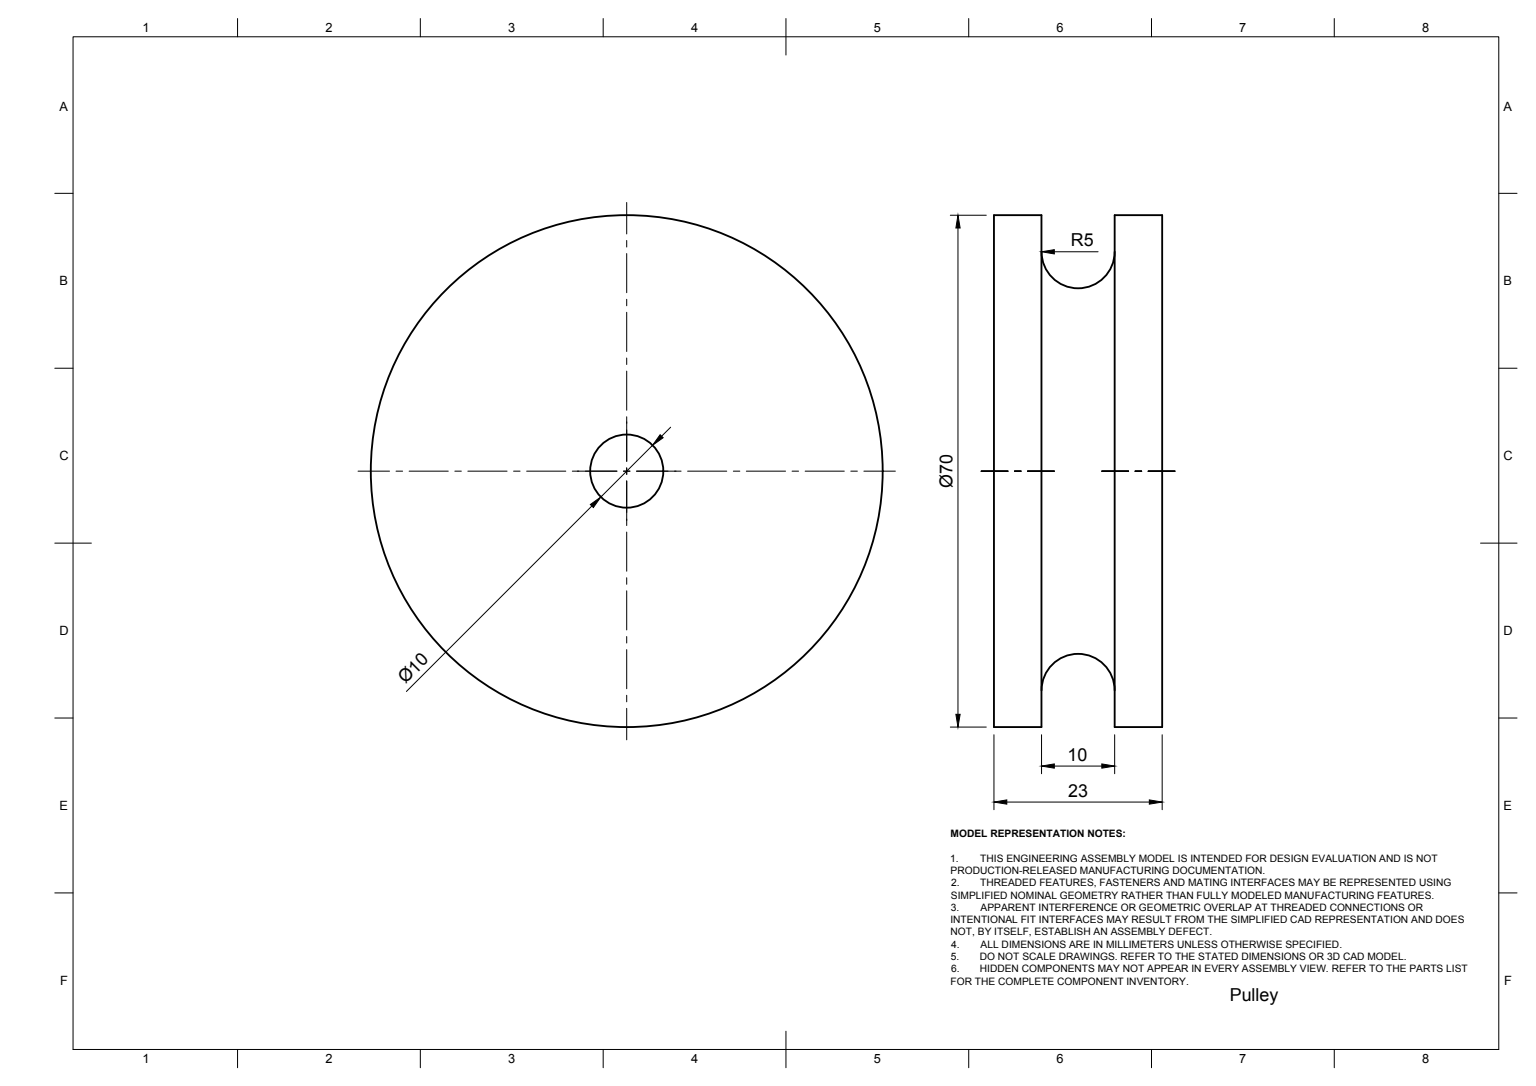
ISO-10303-21;
HEADER;
/* Generated by software containing ST-Developer
 * from STEP Tools, Inc. (www.steptools.com) 
 */

FILE_DESCRIPTION(
/* description */ (''),
/* implementation_level */ '2;1');

FILE_NAME(
/* name */ 'Pulley.step',
/* time_stamp */ '2026-10-07T11:02:43-07:00',
/* author */ (''),
/* organization */ (''),
/* preprocessor_version */ 'ST-DEVELOPER v20.2',
/* originating_system */ 'Autodesk Translation Framework v15.15.0.0',
/* authorisation */ '');

FILE_SCHEMA (('AUTOMOTIVE_DESIGN { 1 0 10303 214 3 1 1 }'));
ENDSEC;

DATA;
#10=MECHANICAL_DESIGN_GEOMETRIC_PRESENTATION_REPRESENTATION('',(#68),#5505);
#51=TOROIDAL_SURFACE('',#3505,30.,5.);
#54=SHAPE_REPRESENTATION_RELATIONSHIP('SRR','None',#5539,#61);
#61=ADVANCED_BREP_SHAPE_REPRESENTATION('',(#75),#5500);
#68=STYLED_ITEM('',(#5583),#75);
#75=MANIFOLD_SOLID_BREP('Body1',#3295);
#98=FACE_BOUND('',#504,.T.);
#99=FACE_BOUND('',#507,.T.);
#100=FACE_BOUND('',#510,.T.);
#101=FACE_BOUND('',#513,.T.);
#129=CYLINDRICAL_SURFACE('',#3496,5.);
#130=CYLINDRICAL_SURFACE('',#3501,35.);
#131=CYLINDRICAL_SURFACE('',#3510,35.);
#185=CIRCLE('',#3497,5.);
#186=CIRCLE('',#3498,5.);
#187=CIRCLE('',#3500,35.);
#188=CIRCLE('',#3502,35.);
#189=CIRCLE('',#3504,30.);
#190=CIRCLE('',#3506,5.);
#191=CIRCLE('',#3507,30.);
#192=CIRCLE('',#3509,35.);
#193=CIRCLE('',#3511,35.);
#318=FACE_OUTER_BOUND('',#502,.T.);
#319=FACE_OUTER_BOUND('',#503,.T.);
#320=FACE_OUTER_BOUND('',#505,.T.);
#321=FACE_OUTER_BOUND('',#506,.T.);
#322=FACE_OUTER_BOUND('',#508,.T.);
#323=FACE_OUTER_BOUND('',#509,.T.);
#324=FACE_OUTER_BOUND('',#511,.T.);
#325=FACE_OUTER_BOUND('',#512,.T.);
#502=EDGE_LOOP('',(#2576,#2577,#2578,#2579));
#503=EDGE_LOOP('',(#2580));
#504=EDGE_LOOP('',(#2581));
#505=EDGE_LOOP('',(#2582,#2583,#2584,#2585));
#506=EDGE_LOOP('',(#2586));
#507=EDGE_LOOP('',(#2587));
#508=EDGE_LOOP('',(#2588,#2589,#2590,#2591));
#509=EDGE_LOOP('',(#2592));
#510=EDGE_LOOP('',(#2593));
#511=EDGE_LOOP('',(#2594,#2595,#2596,#2597));
#512=EDGE_LOOP('',(#2598));
#513=EDGE_LOOP('',(#2599));
#809=LINE('',#5039,#1179);
#810=LINE('',#5046,#1180);
#811=LINE('',#5060,#1181);
#1179=VECTOR('',#4093,5.);
#1180=VECTOR('',#4102,35.);
#1181=VECTOR('',#4121,35.);
#1501=VERTEX_POINT('',#5036);
#1502=VERTEX_POINT('',#5038);
#1503=VERTEX_POINT('',#5042);
#1504=VERTEX_POINT('',#5045);
#1505=VERTEX_POINT('',#5049);
#1506=VERTEX_POINT('',#5052);
#1507=VERTEX_POINT('',#5056);
#1508=VERTEX_POINT('',#5059);
#1883=EDGE_CURVE('',#1501,#1501,#185,.T.);
#1884=EDGE_CURVE('',#1501,#1502,#809,.T.);
#1885=EDGE_CURVE('',#1502,#1502,#186,.T.);
#1886=EDGE_CURVE('',#1503,#1503,#187,.T.);
#1887=EDGE_CURVE('',#1503,#1504,#810,.T.);
#1888=EDGE_CURVE('',#1504,#1504,#188,.T.);
#1889=EDGE_CURVE('',#1505,#1505,#189,.T.);
#1890=EDGE_CURVE('',#1505,#1506,#190,.T.);
#1891=EDGE_CURVE('',#1506,#1506,#191,.T.);
#1892=EDGE_CURVE('',#1507,#1507,#192,.T.);
#1893=EDGE_CURVE('',#1507,#1508,#811,.T.);
#1894=EDGE_CURVE('',#1508,#1508,#193,.T.);
#2576=ORIENTED_EDGE('',*,*,#1883,.F.);
#2577=ORIENTED_EDGE('',*,*,#1884,.T.);
#2578=ORIENTED_EDGE('',*,*,#1885,.T.);
#2579=ORIENTED_EDGE('',*,*,#1884,.F.);
#2580=ORIENTED_EDGE('',*,*,#1886,.T.);
#2581=ORIENTED_EDGE('',*,*,#1885,.F.);
#2582=ORIENTED_EDGE('',*,*,#1886,.F.);
#2583=ORIENTED_EDGE('',*,*,#1887,.T.);
#2584=ORIENTED_EDGE('',*,*,#1888,.T.);
#2585=ORIENTED_EDGE('',*,*,#1887,.F.);
#2586=ORIENTED_EDGE('',*,*,#1888,.F.);
#2587=ORIENTED_EDGE('',*,*,#1889,.T.);
#2588=ORIENTED_EDGE('',*,*,#1889,.F.);
#2589=ORIENTED_EDGE('',*,*,#1890,.T.);
#2590=ORIENTED_EDGE('',*,*,#1891,.T.);
#2591=ORIENTED_EDGE('',*,*,#1890,.F.);
#2592=ORIENTED_EDGE('',*,*,#1892,.T.);
#2593=ORIENTED_EDGE('',*,*,#1891,.F.);
#2594=ORIENTED_EDGE('',*,*,#1892,.F.);
#2595=ORIENTED_EDGE('',*,*,#1893,.T.);
#2596=ORIENTED_EDGE('',*,*,#1894,.T.);
#2597=ORIENTED_EDGE('',*,*,#1893,.F.);
#2598=ORIENTED_EDGE('',*,*,#1894,.F.);
#2599=ORIENTED_EDGE('',*,*,#1883,.T.);
#3068=PLANE('',#3499);
#3069=PLANE('',#3503);
#3070=PLANE('',#3508);
#3071=PLANE('',#3512);
#3209=ADVANCED_FACE('',(#318),#129,.F.);
#3210=ADVANCED_FACE('',(#319,#98),#3068,.F.);
#3211=ADVANCED_FACE('',(#320),#130,.T.);
#3212=ADVANCED_FACE('',(#321,#99),#3069,.T.);
#3213=ADVANCED_FACE('',(#322),#51,.F.);
#3214=ADVANCED_FACE('',(#323,#100),#3070,.F.);
#3215=ADVANCED_FACE('',(#324),#131,.T.);
#3216=ADVANCED_FACE('',(#325,#101),#3071,.T.);
#3295=CLOSED_SHELL('',(#3209,#3210,#3211,#3212,#3213,#3214,#3215,#3216));
#3495=AXIS2_PLACEMENT_3D('',#5034,#4087,#4088);
#3496=AXIS2_PLACEMENT_3D('',#5035,#4089,#4090);
#3497=AXIS2_PLACEMENT_3D('',#5037,#4091,#4092);
#3498=AXIS2_PLACEMENT_3D('',#5040,#4094,#4095);
#3499=AXIS2_PLACEMENT_3D('',#5041,#4096,#4097);
#3500=AXIS2_PLACEMENT_3D('',#5043,#4098,#4099);
#3501=AXIS2_PLACEMENT_3D('',#5044,#4100,#4101);
#3502=AXIS2_PLACEMENT_3D('',#5047,#4103,#4104);
#3503=AXIS2_PLACEMENT_3D('',#5048,#4105,#4106);
#3504=AXIS2_PLACEMENT_3D('',#5050,#4107,#4108);
#3505=AXIS2_PLACEMENT_3D('',#5051,#4109,#4110);
#3506=AXIS2_PLACEMENT_3D('',#5053,#4111,#4112);
#3507=AXIS2_PLACEMENT_3D('',#5054,#4113,#4114);
#3508=AXIS2_PLACEMENT_3D('',#5055,#4115,#4116);
#3509=AXIS2_PLACEMENT_3D('',#5057,#4117,#4118);
#3510=AXIS2_PLACEMENT_3D('',#5058,#4119,#4120);
#3511=AXIS2_PLACEMENT_3D('',#5061,#4122,#4123);
#3512=AXIS2_PLACEMENT_3D('',#5062,#4124,#4125);
#4087=DIRECTION('axis',(0.,0.,1.));
#4088=DIRECTION('refdir',(1.,0.,0.));
#4089=DIRECTION('center_axis',(0.,0.,-1.));
#4090=DIRECTION('ref_axis',(-1.,0.,0.));
#4091=DIRECTION('center_axis',(0.,0.,-1.));
#4092=DIRECTION('ref_axis',(-1.,0.,0.));
#4093=DIRECTION('',(0.,0.,-1.));
#4094=DIRECTION('center_axis',(0.,0.,-1.));
#4095=DIRECTION('ref_axis',(-1.,0.,0.));
#4096=DIRECTION('center_axis',(0.,0.,1.));
#4097=DIRECTION('ref_axis',(1.,0.,0.));
#4098=DIRECTION('center_axis',(0.,0.,-1.));
#4099=DIRECTION('ref_axis',(-1.,0.,0.));
#4100=DIRECTION('center_axis',(0.,0.,-1.));
#4101=DIRECTION('ref_axis',(-1.,0.,0.));
#4102=DIRECTION('',(0.,0.,1.));
#4103=DIRECTION('center_axis',(0.,0.,-1.));
#4104=DIRECTION('ref_axis',(-1.,0.,0.));
#4105=DIRECTION('center_axis',(0.,0.,1.));
#4106=DIRECTION('ref_axis',(1.,0.,0.));
#4107=DIRECTION('center_axis',(0.,0.,-1.));
#4108=DIRECTION('ref_axis',(-1.,0.,0.));
#4109=DIRECTION('center_axis',(0.,0.,-1.));
#4110=DIRECTION('ref_axis',(-1.,0.,0.));
#4111=DIRECTION('center_axis',(0.,1.,0.));
#4112=DIRECTION('ref_axis',(1.,0.,0.));
#4113=DIRECTION('center_axis',(0.,0.,-1.));
#4114=DIRECTION('ref_axis',(-1.,0.,0.));
#4115=DIRECTION('center_axis',(0.,0.,1.));
#4116=DIRECTION('ref_axis',(1.,0.,0.));
#4117=DIRECTION('center_axis',(0.,0.,-1.));
#4118=DIRECTION('ref_axis',(-1.,0.,0.));
#4119=DIRECTION('center_axis',(0.,0.,-1.));
#4120=DIRECTION('ref_axis',(-1.,0.,0.));
#4121=DIRECTION('',(0.,0.,1.));
#4122=DIRECTION('center_axis',(0.,0.,-1.));
#4123=DIRECTION('ref_axis',(-1.,0.,0.));
#4124=DIRECTION('center_axis',(0.,0.,1.));
#4125=DIRECTION('ref_axis',(1.,0.,0.));
#5034=CARTESIAN_POINT('',(0.,0.,0.));
#5035=CARTESIAN_POINT('Origin',(375.,-72.5,0.));
#5036=CARTESIAN_POINT('',(380.,-72.5,11.5));
#5037=CARTESIAN_POINT('Origin',(375.,-72.5,11.5));
#5038=CARTESIAN_POINT('',(380.,-72.5,-11.5));
#5039=CARTESIAN_POINT('',(380.,-72.5,0.));
#5040=CARTESIAN_POINT('Origin',(375.,-72.5,-11.5));
#5041=CARTESIAN_POINT('Origin',(375.,-92.5,-11.5));
#5042=CARTESIAN_POINT('',(410.,-72.5,-11.5));
#5043=CARTESIAN_POINT('Origin',(375.,-72.5,-11.5));
#5044=CARTESIAN_POINT('Origin',(375.,-72.5,0.));
#5045=CARTESIAN_POINT('',(410.,-72.5,-5.));
#5046=CARTESIAN_POINT('',(410.,-72.5,0.));
#5047=CARTESIAN_POINT('Origin',(375.,-72.5,-5.));
#5048=CARTESIAN_POINT('Origin',(375.,-105.,-5.));
#5049=CARTESIAN_POINT('',(405.,-72.5,-5.));
#5050=CARTESIAN_POINT('Origin',(375.,-72.5,-5.));
#5051=CARTESIAN_POINT('Origin',(375.,-72.5,-9.65792954036421E-15));
#5052=CARTESIAN_POINT('',(405.,-72.5,5.));
#5053=CARTESIAN_POINT('Origin',(405.,-72.5,-9.65792954036421E-15));
#5054=CARTESIAN_POINT('Origin',(375.,-72.5,5.));
#5055=CARTESIAN_POINT('Origin',(375.,-105.,5.));
#5056=CARTESIAN_POINT('',(410.,-72.5,5.));
#5057=CARTESIAN_POINT('Origin',(375.,-72.5,5.));
#5058=CARTESIAN_POINT('Origin',(375.,-72.5,0.));
#5059=CARTESIAN_POINT('',(410.,-72.5,11.5));
#5060=CARTESIAN_POINT('',(410.,-72.5,0.));
#5061=CARTESIAN_POINT('Origin',(375.,-72.5,11.5));
#5062=CARTESIAN_POINT('Origin',(375.,-92.5,11.5));
#5491=UNCERTAINTY_MEASURE_WITH_UNIT(LENGTH_MEASURE(0.01),#5506,
'DISTANCE_ACCURACY_VALUE',
'Maximum model space distance between geometric entities at asserted c
onnectivities');
#5496=UNCERTAINTY_MEASURE_WITH_UNIT(LENGTH_MEASURE(0.01),#5506,
'DISTANCE_ACCURACY_VALUE',
'Maximum model space distance between geometric entities at asserted c
onnectivities');
#5500=(
GEOMETRIC_REPRESENTATION_CONTEXT(3)
GLOBAL_UNCERTAINTY_ASSIGNED_CONTEXT((#5491))
GLOBAL_UNIT_ASSIGNED_CONTEXT((#5506,#5508,#5509))
REPRESENTATION_CONTEXT('','3D')
);
#5505=(
GEOMETRIC_REPRESENTATION_CONTEXT(3)
GLOBAL_UNCERTAINTY_ASSIGNED_CONTEXT((#5496))
GLOBAL_UNIT_ASSIGNED_CONTEXT((#5506,#5508,#5509))
REPRESENTATION_CONTEXT('','3D')
);
#5506=(
LENGTH_UNIT()
NAMED_UNIT(*)
SI_UNIT(.MILLI.,.METRE.)
);
#5508=(
NAMED_UNIT(*)
PLANE_ANGLE_UNIT()
SI_UNIT($,.RADIAN.)
);
#5509=(
NAMED_UNIT(*)
SI_UNIT($,.STERADIAN.)
SOLID_ANGLE_UNIT()
);
#5513=SHAPE_DEFINITION_REPRESENTATION(#5521,#5539);
#5521=PRODUCT_DEFINITION_SHAPE('',$,#5548);
#5539=SHAPE_REPRESENTATION('',(#3495),#5500);
#5544=PRODUCT_DEFINITION_CONTEXT('part definition',#5570,'design');
#5548=PRODUCT_DEFINITION('2026-10-07-17-01-32-968','Pulley',#5556,#5544);
#5556=PRODUCT_DEFINITION_FORMATION('',$,#5575);
#5570=APPLICATION_CONTEXT(
'Core Data for Automotive Mechanical Design Process');
#5571=PRODUCT_CONTEXT('part definition',#5570,'mechanical');
#5575=PRODUCT('2026-10-07-17-01-32-968','Pulley','20pcs-pulley',(#5571));
#5583=PRESENTATION_STYLE_ASSIGNMENT((#5591));
#5591=SURFACE_STYLE_USAGE(.BOTH.,#5599);
#5599=SURFACE_SIDE_STYLE('',(#5607));
#5607=SURFACE_STYLE_FILL_AREA(#5615);
#5615=FILL_AREA_STYLE('Opaque(59,97,180)',(#5623));
#5623=FILL_AREA_STYLE_COLOUR('Opaque(59,97,180)',#5631);
#5631=COLOUR_RGB('Opaque(59,97,180)', 0.31764706, 0.68627451, 0.89019608);
ENDSEC;
END-ISO-10303-21;
